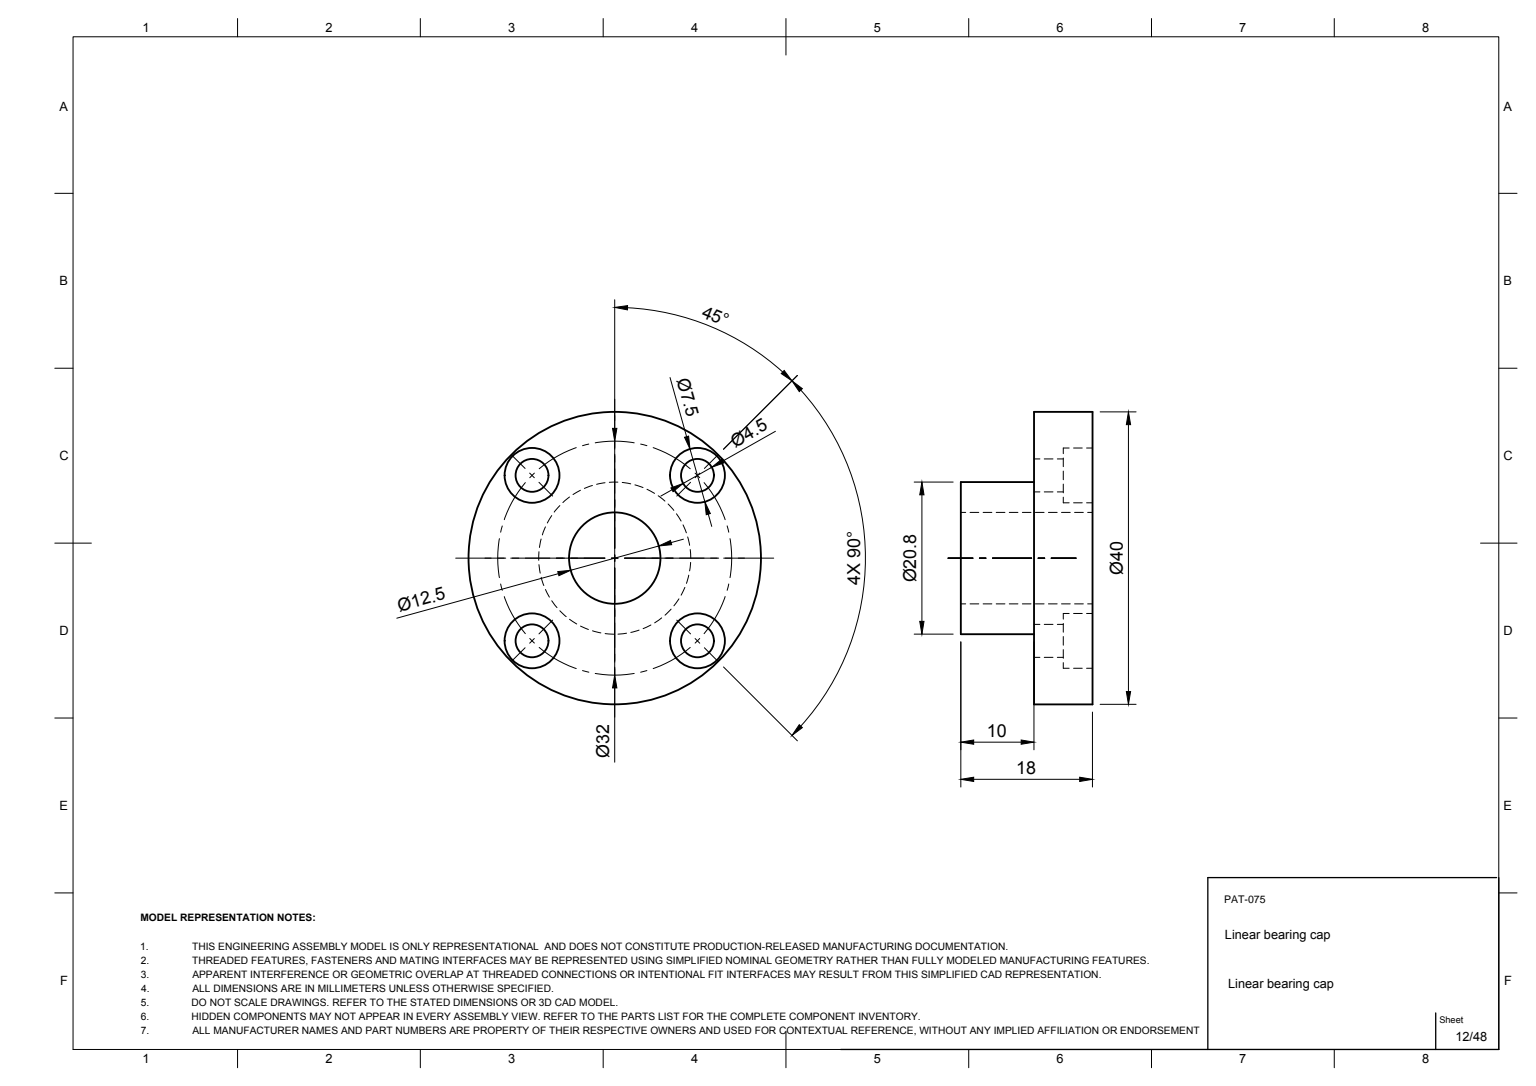
ISO-10303-21;
HEADER;
/* Generated by software containing ST-Developer
 * from STEP Tools, Inc. (www.steptools.com) 
 */

FILE_DESCRIPTION(
/* description */ ('Over-Centre Plunger Toggle Clamp on Slotted Fixture Frame'),
/* implementation_level */ '2;1');

FILE_NAME(
/* name */ 
'Linear bearing cap.step',
/* time_stamp */ '2026-10-28T03:23:24-07:00',
/* author */ (''),
/* organization */ (''),
/* preprocessor_version */ 'ST-DEVELOPER v20.2',
/* originating_system */ 'Autodesk Translation Framework v15.17.0.0',
/* authorisation */ '');

FILE_SCHEMA (('AUTOMOTIVE_DESIGN { 1 0 10303 214 3 1 1 }'));
ENDSEC;

DATA;
#10=MECHANICAL_DESIGN_GEOMETRIC_PRESENTATION_REPRESENTATION('',(#520),#15212);
#436=SHAPE_REPRESENTATION_RELATIONSHIP('SRR','None',#15410,#478);
#478=ADVANCED_BREP_SHAPE_REPRESENTATION('',(#571),#15172);
#520=STYLED_ITEM('',(#15719),#571);
#571=MANIFOLD_SOLID_BREP('Body1',#8252);
#693=FACE_BOUND('',#1755,.T.);
#694=FACE_BOUND('',#1758,.T.);
#695=FACE_BOUND('',#1761,.T.);
#696=FACE_BOUND('',#1764,.T.);
#697=FACE_BOUND('',#1771,.T.);
#698=FACE_BOUND('',#1775,.T.);
#699=FACE_BOUND('',#1776,.T.);
#700=FACE_BOUND('',#1777,.T.);
#701=FACE_BOUND('',#1778,.T.);
#702=FACE_BOUND('',#1779,.T.);
#703=FACE_BOUND('',#1781,.T.);
#704=FACE_BOUND('',#1782,.T.);
#705=FACE_BOUND('',#1783,.T.);
#706=FACE_BOUND('',#1784,.T.);
#707=FACE_BOUND('',#1785,.T.);
#833=PLANE('',#8970);
#834=PLANE('',#8975);
#835=PLANE('',#8980);
#836=PLANE('',#8985);
#837=PLANE('',#8998);
#838=PLANE('',#9005);
#839=PLANE('',#9006);
#1185=FACE_OUTER_BOUND('',#1753,.T.);
#1186=FACE_OUTER_BOUND('',#1754,.T.);
#1187=FACE_OUTER_BOUND('',#1756,.T.);
#1188=FACE_OUTER_BOUND('',#1757,.T.);
#1189=FACE_OUTER_BOUND('',#1759,.T.);
#1190=FACE_OUTER_BOUND('',#1760,.T.);
#1191=FACE_OUTER_BOUND('',#1762,.T.);
#1192=FACE_OUTER_BOUND('',#1763,.T.);
#1193=FACE_OUTER_BOUND('',#1765,.T.);
#1194=FACE_OUTER_BOUND('',#1766,.T.);
#1195=FACE_OUTER_BOUND('',#1767,.T.);
#1196=FACE_OUTER_BOUND('',#1768,.T.);
#1197=FACE_OUTER_BOUND('',#1769,.T.);
#1198=FACE_OUTER_BOUND('',#1770,.T.);
#1199=FACE_OUTER_BOUND('',#1772,.T.);
#1200=FACE_OUTER_BOUND('',#1773,.T.);
#1201=FACE_OUTER_BOUND('',#1774,.T.);
#1202=FACE_OUTER_BOUND('',#1780,.T.);
#1753=EDGE_LOOP('',(#6025,#6026,#6027,#6028));
#1754=EDGE_LOOP('',(#6029));
#1755=EDGE_LOOP('',(#6030));
#1756=EDGE_LOOP('',(#6031,#6032,#6033,#6034));
#1757=EDGE_LOOP('',(#6035));
#1758=EDGE_LOOP('',(#6036));
#1759=EDGE_LOOP('',(#6037,#6038,#6039,#6040));
#1760=EDGE_LOOP('',(#6041));
#1761=EDGE_LOOP('',(#6042));
#1762=EDGE_LOOP('',(#6043,#6044,#6045,#6046));
#1763=EDGE_LOOP('',(#6047));
#1764=EDGE_LOOP('',(#6048));
#1765=EDGE_LOOP('',(#6049,#6050,#6051,#6052));
#1766=EDGE_LOOP('',(#6053,#6054,#6055,#6056));
#1767=EDGE_LOOP('',(#6057,#6058,#6059,#6060));
#1768=EDGE_LOOP('',(#6061,#6062,#6063,#6064));
#1769=EDGE_LOOP('',(#6065,#6066,#6067,#6068));
#1770=EDGE_LOOP('',(#6069));
#1771=EDGE_LOOP('',(#6070));
#1772=EDGE_LOOP('',(#6071,#6072,#6073,#6074));
#1773=EDGE_LOOP('',(#6075,#6076,#6077,#6078));
#1774=EDGE_LOOP('',(#6079));
#1775=EDGE_LOOP('',(#6080));
#1776=EDGE_LOOP('',(#6081));
#1777=EDGE_LOOP('',(#6082));
#1778=EDGE_LOOP('',(#6083));
#1779=EDGE_LOOP('',(#6084));
#1780=EDGE_LOOP('',(#6085));
#1781=EDGE_LOOP('',(#6086));
#1782=EDGE_LOOP('',(#6087));
#1783=EDGE_LOOP('',(#6088));
#1784=EDGE_LOOP('',(#6089));
#1785=EDGE_LOOP('',(#6090));
#2363=LINE('',#12858,#2993);
#2364=LINE('',#12867,#2994);
#2365=LINE('',#12876,#2995);
#2366=LINE('',#12885,#2996);
#2367=LINE('',#12893,#2997);
#2368=LINE('',#12897,#2998);
#2369=LINE('',#12901,#2999);
#2370=LINE('',#12905,#3000);
#2371=LINE('',#12910,#3001);
#2372=LINE('',#12918,#3002);
#2373=LINE('',#12923,#3003);
#2993=VECTOR('',#10298,0.375);
#2994=VECTOR('',#10309,0.375);
#2995=VECTOR('',#10320,0.375);
#2996=VECTOR('',#10331,0.375);
#2997=VECTOR('',#10342,0.225);
#2998=VECTOR('',#10347,0.225);
#2999=VECTOR('',#10352,0.225);
#3000=VECTOR('',#10357,0.225);
#3001=VECTOR('',#10362,1.04);
#3002=VECTOR('',#10373,0.625);
#3003=VECTOR('',#10378,2.);
#3587=CIRCLE('',#8968,0.375);
#3588=CIRCLE('',#8969,0.375);
#3589=CIRCLE('',#8971,0.225);
#3590=CIRCLE('',#8973,0.375);
#3591=CIRCLE('',#8974,0.375);
#3592=CIRCLE('',#8976,0.225);
#3593=CIRCLE('',#8978,0.375);
#3594=CIRCLE('',#8979,0.375);
#3595=CIRCLE('',#8981,0.225);
#3596=CIRCLE('',#8983,0.375);
#3597=CIRCLE('',#8984,0.375);
#3598=CIRCLE('',#8986,0.225);
#3599=CIRCLE('',#8988,0.225);
#3600=CIRCLE('',#8990,0.225);
#3601=CIRCLE('',#8992,0.225);
#3602=CIRCLE('',#8994,0.225);
#3603=CIRCLE('',#8996,1.04);
#3604=CIRCLE('',#8997,1.04);
#3605=CIRCLE('',#8999,0.625);
#3606=CIRCLE('',#9001,0.625);
#3607=CIRCLE('',#9003,2.);
#3608=CIRCLE('',#9004,2.);
#4011=VERTEX_POINT('',#12855);
#4012=VERTEX_POINT('',#12857);
#4013=VERTEX_POINT('',#12861);
#4014=VERTEX_POINT('',#12864);
#4015=VERTEX_POINT('',#12866);
#4016=VERTEX_POINT('',#12870);
#4017=VERTEX_POINT('',#12873);
#4018=VERTEX_POINT('',#12875);
#4019=VERTEX_POINT('',#12879);
#4020=VERTEX_POINT('',#12882);
#4021=VERTEX_POINT('',#12884);
#4022=VERTEX_POINT('',#12888);
#4023=VERTEX_POINT('',#12891);
#4024=VERTEX_POINT('',#12895);
#4025=VERTEX_POINT('',#12899);
#4026=VERTEX_POINT('',#12903);
#4027=VERTEX_POINT('',#12907);
#4028=VERTEX_POINT('',#12909);
#4029=VERTEX_POINT('',#12913);
#4030=VERTEX_POINT('',#12916);
#4031=VERTEX_POINT('',#12920);
#4032=VERTEX_POINT('',#12922);
#4773=EDGE_CURVE('',#4011,#4011,#3587,.T.);
#4774=EDGE_CURVE('',#4011,#4012,#2363,.T.);
#4775=EDGE_CURVE('',#4012,#4012,#3588,.T.);
#4776=EDGE_CURVE('',#4013,#4013,#3589,.T.);
#4777=EDGE_CURVE('',#4014,#4014,#3590,.T.);
#4778=EDGE_CURVE('',#4014,#4015,#2364,.T.);
#4779=EDGE_CURVE('',#4015,#4015,#3591,.T.);
#4780=EDGE_CURVE('',#4016,#4016,#3592,.T.);
#4781=EDGE_CURVE('',#4017,#4017,#3593,.T.);
#4782=EDGE_CURVE('',#4017,#4018,#2365,.T.);
#4783=EDGE_CURVE('',#4018,#4018,#3594,.T.);
#4784=EDGE_CURVE('',#4019,#4019,#3595,.T.);
#4785=EDGE_CURVE('',#4020,#4020,#3596,.T.);
#4786=EDGE_CURVE('',#4020,#4021,#2366,.T.);
#4787=EDGE_CURVE('',#4021,#4021,#3597,.T.);
#4788=EDGE_CURVE('',#4022,#4022,#3598,.T.);
#4789=EDGE_CURVE('',#4023,#4023,#3599,.T.);
#4790=EDGE_CURVE('',#4023,#4013,#2367,.T.);
#4791=EDGE_CURVE('',#4024,#4024,#3600,.T.);
#4792=EDGE_CURVE('',#4024,#4016,#2368,.T.);
#4793=EDGE_CURVE('',#4025,#4025,#3601,.T.);
#4794=EDGE_CURVE('',#4025,#4019,#2369,.T.);
#4795=EDGE_CURVE('',#4026,#4026,#3602,.T.);
#4796=EDGE_CURVE('',#4026,#4022,#2370,.T.);
#4797=EDGE_CURVE('',#4027,#4027,#3603,.T.);
#4798=EDGE_CURVE('',#4027,#4028,#2371,.T.);
#4799=EDGE_CURVE('',#4028,#4028,#3604,.T.);
#4800=EDGE_CURVE('',#4029,#4029,#3605,.T.);
#4801=EDGE_CURVE('',#4030,#4030,#3606,.T.);
#4802=EDGE_CURVE('',#4030,#4029,#2372,.T.);
#4803=EDGE_CURVE('',#4031,#4031,#3607,.T.);
#4804=EDGE_CURVE('',#4031,#4032,#2373,.T.);
#4805=EDGE_CURVE('',#4032,#4032,#3608,.T.);
#6025=ORIENTED_EDGE('',*,*,#4773,.F.);
#6026=ORIENTED_EDGE('',*,*,#4774,.T.);
#6027=ORIENTED_EDGE('',*,*,#4775,.F.);
#6028=ORIENTED_EDGE('',*,*,#4774,.F.);
#6029=ORIENTED_EDGE('',*,*,#4773,.T.);
#6030=ORIENTED_EDGE('',*,*,#4776,.F.);
#6031=ORIENTED_EDGE('',*,*,#4777,.F.);
#6032=ORIENTED_EDGE('',*,*,#4778,.T.);
#6033=ORIENTED_EDGE('',*,*,#4779,.F.);
#6034=ORIENTED_EDGE('',*,*,#4778,.F.);
#6035=ORIENTED_EDGE('',*,*,#4777,.T.);
#6036=ORIENTED_EDGE('',*,*,#4780,.F.);
#6037=ORIENTED_EDGE('',*,*,#4781,.F.);
#6038=ORIENTED_EDGE('',*,*,#4782,.T.);
#6039=ORIENTED_EDGE('',*,*,#4783,.F.);
#6040=ORIENTED_EDGE('',*,*,#4782,.F.);
#6041=ORIENTED_EDGE('',*,*,#4781,.T.);
#6042=ORIENTED_EDGE('',*,*,#4784,.F.);
#6043=ORIENTED_EDGE('',*,*,#4785,.F.);
#6044=ORIENTED_EDGE('',*,*,#4786,.T.);
#6045=ORIENTED_EDGE('',*,*,#4787,.F.);
#6046=ORIENTED_EDGE('',*,*,#4786,.F.);
#6047=ORIENTED_EDGE('',*,*,#4785,.T.);
#6048=ORIENTED_EDGE('',*,*,#4788,.F.);
#6049=ORIENTED_EDGE('',*,*,#4789,.F.);
#6050=ORIENTED_EDGE('',*,*,#4790,.T.);
#6051=ORIENTED_EDGE('',*,*,#4776,.T.);
#6052=ORIENTED_EDGE('',*,*,#4790,.F.);
#6053=ORIENTED_EDGE('',*,*,#4791,.F.);
#6054=ORIENTED_EDGE('',*,*,#4792,.T.);
#6055=ORIENTED_EDGE('',*,*,#4780,.T.);
#6056=ORIENTED_EDGE('',*,*,#4792,.F.);
#6057=ORIENTED_EDGE('',*,*,#4793,.F.);
#6058=ORIENTED_EDGE('',*,*,#4794,.T.);
#6059=ORIENTED_EDGE('',*,*,#4784,.T.);
#6060=ORIENTED_EDGE('',*,*,#4794,.F.);
#6061=ORIENTED_EDGE('',*,*,#4795,.F.);
#6062=ORIENTED_EDGE('',*,*,#4796,.T.);
#6063=ORIENTED_EDGE('',*,*,#4788,.T.);
#6064=ORIENTED_EDGE('',*,*,#4796,.F.);
#6065=ORIENTED_EDGE('',*,*,#4797,.F.);
#6066=ORIENTED_EDGE('',*,*,#4798,.T.);
#6067=ORIENTED_EDGE('',*,*,#4799,.T.);
#6068=ORIENTED_EDGE('',*,*,#4798,.F.);
#6069=ORIENTED_EDGE('',*,*,#4799,.F.);
#6070=ORIENTED_EDGE('',*,*,#4800,.F.);
#6071=ORIENTED_EDGE('',*,*,#4801,.F.);
#6072=ORIENTED_EDGE('',*,*,#4802,.T.);
#6073=ORIENTED_EDGE('',*,*,#4800,.T.);
#6074=ORIENTED_EDGE('',*,*,#4802,.F.);
#6075=ORIENTED_EDGE('',*,*,#4803,.F.);
#6076=ORIENTED_EDGE('',*,*,#4804,.T.);
#6077=ORIENTED_EDGE('',*,*,#4805,.T.);
#6078=ORIENTED_EDGE('',*,*,#4804,.F.);
#6079=ORIENTED_EDGE('',*,*,#4803,.T.);
#6080=ORIENTED_EDGE('',*,*,#4801,.T.);
#6081=ORIENTED_EDGE('',*,*,#4787,.T.);
#6082=ORIENTED_EDGE('',*,*,#4783,.T.);
#6083=ORIENTED_EDGE('',*,*,#4779,.T.);
#6084=ORIENTED_EDGE('',*,*,#4775,.T.);
#6085=ORIENTED_EDGE('',*,*,#4805,.F.);
#6086=ORIENTED_EDGE('',*,*,#4797,.T.);
#6087=ORIENTED_EDGE('',*,*,#4795,.T.);
#6088=ORIENTED_EDGE('',*,*,#4793,.T.);
#6089=ORIENTED_EDGE('',*,*,#4791,.T.);
#6090=ORIENTED_EDGE('',*,*,#4789,.T.);
#7665=CYLINDRICAL_SURFACE('',#8967,0.375);
#7666=CYLINDRICAL_SURFACE('',#8972,0.375);
#7667=CYLINDRICAL_SURFACE('',#8977,0.375);
#7668=CYLINDRICAL_SURFACE('',#8982,0.375);
#7669=CYLINDRICAL_SURFACE('',#8987,0.225);
#7670=CYLINDRICAL_SURFACE('',#8989,0.225);
#7671=CYLINDRICAL_SURFACE('',#8991,0.225);
#7672=CYLINDRICAL_SURFACE('',#8993,0.225);
#7673=CYLINDRICAL_SURFACE('',#8995,1.04);
#7674=CYLINDRICAL_SURFACE('',#9000,0.625);
#7675=CYLINDRICAL_SURFACE('',#9002,2.);
#7857=ADVANCED_FACE('',(#1185),#7665,.F.);
#7858=ADVANCED_FACE('',(#1186,#693),#833,.T.);
#7859=ADVANCED_FACE('',(#1187),#7666,.F.);
#7860=ADVANCED_FACE('',(#1188,#694),#834,.T.);
#7861=ADVANCED_FACE('',(#1189),#7667,.F.);
#7862=ADVANCED_FACE('',(#1190,#695),#835,.T.);
#7863=ADVANCED_FACE('',(#1191),#7668,.F.);
#7864=ADVANCED_FACE('',(#1192,#696),#836,.T.);
#7865=ADVANCED_FACE('',(#1193),#7669,.F.);
#7866=ADVANCED_FACE('',(#1194),#7670,.F.);
#7867=ADVANCED_FACE('',(#1195),#7671,.F.);
#7868=ADVANCED_FACE('',(#1196),#7672,.F.);
#7869=ADVANCED_FACE('',(#1197),#7673,.T.);
#7870=ADVANCED_FACE('',(#1198,#697),#837,.F.);
#7871=ADVANCED_FACE('',(#1199),#7674,.F.);
#7872=ADVANCED_FACE('',(#1200),#7675,.T.);
#7873=ADVANCED_FACE('',(#1201,#698,#699,#700,#701,#702),#838,.T.);
#7874=ADVANCED_FACE('',(#1202,#703,#704,#705,#706,#707),#839,.F.);
#8252=CLOSED_SHELL('',(#7857,#7858,#7859,#7860,#7861,#7862,#7863,#7864,
#7865,#7866,#7867,#7868,#7869,#7870,#7871,#7872,#7873,#7874));
#8966=AXIS2_PLACEMENT_3D('',#12853,#10292,#10293);
#8967=AXIS2_PLACEMENT_3D('',#12854,#10294,#10295);
#8968=AXIS2_PLACEMENT_3D('',#12856,#10296,#10297);
#8969=AXIS2_PLACEMENT_3D('',#12859,#10299,#10300);
#8970=AXIS2_PLACEMENT_3D('',#12860,#10301,#10302);
#8971=AXIS2_PLACEMENT_3D('',#12862,#10303,#10304);
#8972=AXIS2_PLACEMENT_3D('',#12863,#10305,#10306);
#8973=AXIS2_PLACEMENT_3D('',#12865,#10307,#10308);
#8974=AXIS2_PLACEMENT_3D('',#12868,#10310,#10311);
#8975=AXIS2_PLACEMENT_3D('',#12869,#10312,#10313);
#8976=AXIS2_PLACEMENT_3D('',#12871,#10314,#10315);
#8977=AXIS2_PLACEMENT_3D('',#12872,#10316,#10317);
#8978=AXIS2_PLACEMENT_3D('',#12874,#10318,#10319);
#8979=AXIS2_PLACEMENT_3D('',#12877,#10321,#10322);
#8980=AXIS2_PLACEMENT_3D('',#12878,#10323,#10324);
#8981=AXIS2_PLACEMENT_3D('',#12880,#10325,#10326);
#8982=AXIS2_PLACEMENT_3D('',#12881,#10327,#10328);
#8983=AXIS2_PLACEMENT_3D('',#12883,#10329,#10330);
#8984=AXIS2_PLACEMENT_3D('',#12886,#10332,#10333);
#8985=AXIS2_PLACEMENT_3D('',#12887,#10334,#10335);
#8986=AXIS2_PLACEMENT_3D('',#12889,#10336,#10337);
#8987=AXIS2_PLACEMENT_3D('',#12890,#10338,#10339);
#8988=AXIS2_PLACEMENT_3D('',#12892,#10340,#10341);
#8989=AXIS2_PLACEMENT_3D('',#12894,#10343,#10344);
#8990=AXIS2_PLACEMENT_3D('',#12896,#10345,#10346);
#8991=AXIS2_PLACEMENT_3D('',#12898,#10348,#10349);
#8992=AXIS2_PLACEMENT_3D('',#12900,#10350,#10351);
#8993=AXIS2_PLACEMENT_3D('',#12902,#10353,#10354);
#8994=AXIS2_PLACEMENT_3D('',#12904,#10355,#10356);
#8995=AXIS2_PLACEMENT_3D('',#12906,#10358,#10359);
#8996=AXIS2_PLACEMENT_3D('',#12908,#10360,#10361);
#8997=AXIS2_PLACEMENT_3D('',#12911,#10363,#10364);
#8998=AXIS2_PLACEMENT_3D('',#12912,#10365,#10366);
#8999=AXIS2_PLACEMENT_3D('',#12914,#10367,#10368);
#9000=AXIS2_PLACEMENT_3D('',#12915,#10369,#10370);
#9001=AXIS2_PLACEMENT_3D('',#12917,#10371,#10372);
#9002=AXIS2_PLACEMENT_3D('',#12919,#10374,#10375);
#9003=AXIS2_PLACEMENT_3D('',#12921,#10376,#10377);
#9004=AXIS2_PLACEMENT_3D('',#12924,#10379,#10380);
#9005=AXIS2_PLACEMENT_3D('',#12925,#10381,#10382);
#9006=AXIS2_PLACEMENT_3D('',#12926,#10383,#10384);
#10292=DIRECTION('axis',(0.,0.,1.));
#10293=DIRECTION('refdir',(1.,0.,0.));
#10294=DIRECTION('center_axis',(0.,0.,1.));
#10295=DIRECTION('ref_axis',(1.,0.,0.));
#10296=DIRECTION('center_axis',(0.,0.,1.));
#10297=DIRECTION('ref_axis',(1.,0.,0.));
#10298=DIRECTION('',(0.,0.,1.));
#10299=DIRECTION('center_axis',(0.,0.,-1.));
#10300=DIRECTION('ref_axis',(1.,0.,0.));
#10301=DIRECTION('center_axis',(0.,0.,1.));
#10302=DIRECTION('ref_axis',(1.,0.,0.));
#10303=DIRECTION('center_axis',(0.,0.,1.));
#10304=DIRECTION('ref_axis',(1.,0.,0.));
#10305=DIRECTION('center_axis',(0.,0.,1.));
#10306=DIRECTION('ref_axis',(1.,0.,0.));
#10307=DIRECTION('center_axis',(0.,0.,1.));
#10308=DIRECTION('ref_axis',(1.,0.,0.));
#10309=DIRECTION('',(0.,0.,1.));
#10310=DIRECTION('center_axis',(0.,0.,-1.));
#10311=DIRECTION('ref_axis',(1.,0.,0.));
#10312=DIRECTION('center_axis',(0.,0.,1.));
#10313=DIRECTION('ref_axis',(1.,0.,0.));
#10314=DIRECTION('center_axis',(0.,0.,1.));
#10315=DIRECTION('ref_axis',(1.,0.,0.));
#10316=DIRECTION('center_axis',(0.,0.,1.));
#10317=DIRECTION('ref_axis',(1.,0.,0.));
#10318=DIRECTION('center_axis',(0.,0.,1.));
#10319=DIRECTION('ref_axis',(1.,0.,0.));
#10320=DIRECTION('',(0.,0.,1.));
#10321=DIRECTION('center_axis',(0.,0.,-1.));
#10322=DIRECTION('ref_axis',(1.,0.,0.));
#10323=DIRECTION('center_axis',(0.,0.,1.));
#10324=DIRECTION('ref_axis',(1.,0.,0.));
#10325=DIRECTION('center_axis',(0.,0.,1.));
#10326=DIRECTION('ref_axis',(1.,0.,0.));
#10327=DIRECTION('center_axis',(0.,0.,1.));
#10328=DIRECTION('ref_axis',(1.,0.,0.));
#10329=DIRECTION('center_axis',(0.,0.,1.));
#10330=DIRECTION('ref_axis',(1.,0.,0.));
#10331=DIRECTION('',(0.,0.,1.));
#10332=DIRECTION('center_axis',(0.,0.,-1.));
#10333=DIRECTION('ref_axis',(1.,0.,0.));
#10334=DIRECTION('center_axis',(0.,0.,1.));
#10335=DIRECTION('ref_axis',(1.,0.,0.));
#10336=DIRECTION('center_axis',(0.,0.,1.));
#10337=DIRECTION('ref_axis',(1.,0.,0.));
#10338=DIRECTION('center_axis',(0.,0.,1.));
#10339=DIRECTION('ref_axis',(1.,0.,0.));
#10340=DIRECTION('center_axis',(0.,0.,1.));
#10341=DIRECTION('ref_axis',(1.,0.,0.));
#10342=DIRECTION('',(0.,0.,1.));
#10343=DIRECTION('center_axis',(0.,0.,1.));
#10344=DIRECTION('ref_axis',(1.,0.,0.));
#10345=DIRECTION('center_axis',(0.,0.,1.));
#10346=DIRECTION('ref_axis',(1.,0.,0.));
#10347=DIRECTION('',(0.,0.,1.));
#10348=DIRECTION('center_axis',(0.,0.,1.));
#10349=DIRECTION('ref_axis',(1.,0.,0.));
#10350=DIRECTION('center_axis',(0.,0.,1.));
#10351=DIRECTION('ref_axis',(1.,0.,0.));
#10352=DIRECTION('',(0.,0.,1.));
#10353=DIRECTION('center_axis',(0.,0.,1.));
#10354=DIRECTION('ref_axis',(1.,0.,0.));
#10355=DIRECTION('center_axis',(0.,0.,1.));
#10356=DIRECTION('ref_axis',(1.,0.,0.));
#10357=DIRECTION('',(0.,0.,1.));
#10358=DIRECTION('center_axis',(0.,0.,1.));
#10359=DIRECTION('ref_axis',(1.,0.,0.));
#10360=DIRECTION('center_axis',(0.,0.,1.));
#10361=DIRECTION('ref_axis',(1.,0.,0.));
#10362=DIRECTION('',(0.,0.,-1.));
#10363=DIRECTION('center_axis',(0.,0.,1.));
#10364=DIRECTION('ref_axis',(1.,0.,0.));
#10365=DIRECTION('center_axis',(0.,0.,1.));
#10366=DIRECTION('ref_axis',(1.,0.,0.));
#10367=DIRECTION('center_axis',(0.,0.,-1.));
#10368=DIRECTION('ref_axis',(1.,0.,0.));
#10369=DIRECTION('center_axis',(0.,0.,1.));
#10370=DIRECTION('ref_axis',(1.,0.,0.));
#10371=DIRECTION('center_axis',(0.,0.,-1.));
#10372=DIRECTION('ref_axis',(1.,0.,0.));
#10373=DIRECTION('',(0.,0.,-1.));
#10374=DIRECTION('center_axis',(0.,0.,1.));
#10375=DIRECTION('ref_axis',(1.,0.,0.));
#10376=DIRECTION('center_axis',(0.,0.,1.));
#10377=DIRECTION('ref_axis',(1.,0.,0.));
#10378=DIRECTION('',(0.,0.,-1.));
#10379=DIRECTION('center_axis',(0.,0.,1.));
#10380=DIRECTION('ref_axis',(1.,0.,0.));
#10381=DIRECTION('center_axis',(0.,0.,1.));
#10382=DIRECTION('ref_axis',(1.,0.,0.));
#10383=DIRECTION('center_axis',(0.,0.,1.));
#10384=DIRECTION('ref_axis',(1.,0.,0.));
#12853=CARTESIAN_POINT('',(0.,0.,0.));
#12854=CARTESIAN_POINT('Origin',(-1.13137084989848,-1.13137084989848,16.9));
#12855=CARTESIAN_POINT('',(-1.50637084989848,-1.13137084989848,16.9));
#12856=CARTESIAN_POINT('Origin',(-1.13137084989848,-1.13137084989848,16.9));
#12857=CARTESIAN_POINT('',(-1.50637084989848,-1.13137084989848,17.3));
#12858=CARTESIAN_POINT('',(-1.50637084989848,-1.13137084989848,16.9));
#12859=CARTESIAN_POINT('Origin',(-1.13137084989848,-1.13137084989848,17.3));
#12860=CARTESIAN_POINT('Origin',(-1.13137084989848,-1.13137084989848,16.9));
#12861=CARTESIAN_POINT('',(-1.35637084989848,-1.13137084989848,16.9));
#12862=CARTESIAN_POINT('Origin',(-1.13137084989848,-1.13137084989848,16.9));
#12863=CARTESIAN_POINT('Origin',(-1.13137084989848,1.13137084989848,16.9));
#12864=CARTESIAN_POINT('',(-1.50637084989848,1.13137084989848,16.9));
#12865=CARTESIAN_POINT('Origin',(-1.13137084989848,1.13137084989848,16.9));
#12866=CARTESIAN_POINT('',(-1.50637084989848,1.13137084989848,17.3));
#12867=CARTESIAN_POINT('',(-1.50637084989848,1.13137084989848,16.9));
#12868=CARTESIAN_POINT('Origin',(-1.13137084989848,1.13137084989848,17.3));
#12869=CARTESIAN_POINT('Origin',(-1.13137084989848,1.13137084989848,16.9));
#12870=CARTESIAN_POINT('',(-1.35637084989848,1.13137084989848,16.9));
#12871=CARTESIAN_POINT('Origin',(-1.13137084989848,1.13137084989848,16.9));
#12872=CARTESIAN_POINT('Origin',(1.13137084989848,1.13137084989848,16.9));
#12873=CARTESIAN_POINT('',(0.756370849898476,1.13137084989848,16.9));
#12874=CARTESIAN_POINT('Origin',(1.13137084989848,1.13137084989848,16.9));
#12875=CARTESIAN_POINT('',(0.756370849898476,1.13137084989848,17.3));
#12876=CARTESIAN_POINT('',(0.756370849898476,1.13137084989848,16.9));
#12877=CARTESIAN_POINT('Origin',(1.13137084989848,1.13137084989848,17.3));
#12878=CARTESIAN_POINT('Origin',(1.13137084989848,1.13137084989848,16.9));
#12879=CARTESIAN_POINT('',(0.906370849898476,1.13137084989848,16.9));
#12880=CARTESIAN_POINT('Origin',(1.13137084989848,1.13137084989848,16.9));
#12881=CARTESIAN_POINT('Origin',(1.13137084989848,-1.13137084989848,16.9));
#12882=CARTESIAN_POINT('',(0.756370849898476,-1.13137084989848,16.9));
#12883=CARTESIAN_POINT('Origin',(1.13137084989848,-1.13137084989848,16.9));
#12884=CARTESIAN_POINT('',(0.756370849898476,-1.13137084989848,17.3));
#12885=CARTESIAN_POINT('',(0.756370849898476,-1.13137084989848,16.9));
#12886=CARTESIAN_POINT('Origin',(1.13137084989848,-1.13137084989848,17.3));
#12887=CARTESIAN_POINT('Origin',(1.13137084989848,-1.13137084989848,16.9));
#12888=CARTESIAN_POINT('',(0.906370849898476,-1.13137084989848,16.9));
#12889=CARTESIAN_POINT('Origin',(1.13137084989848,-1.13137084989848,16.9));
#12890=CARTESIAN_POINT('Origin',(-1.13137084989848,-1.13137084989848,16.4));
#12891=CARTESIAN_POINT('',(-1.35637084989848,-1.13137084989848,16.5));
#12892=CARTESIAN_POINT('Origin',(-1.13137084989848,-1.13137084989848,16.5));
#12893=CARTESIAN_POINT('',(-1.35637084989848,-1.13137084989848,16.4));
#12894=CARTESIAN_POINT('Origin',(-1.13137084989848,1.13137084989848,16.4));
#12895=CARTESIAN_POINT('',(-1.35637084989848,1.13137084989848,16.5));
#12896=CARTESIAN_POINT('Origin',(-1.13137084989848,1.13137084989848,16.5));
#12897=CARTESIAN_POINT('',(-1.35637084989848,1.13137084989848,16.4));
#12898=CARTESIAN_POINT('Origin',(1.13137084989848,1.13137084989848,16.4));
#12899=CARTESIAN_POINT('',(0.906370849898476,1.13137084989848,16.5));
#12900=CARTESIAN_POINT('Origin',(1.13137084989848,1.13137084989848,16.5));
#12901=CARTESIAN_POINT('',(0.906370849898476,1.13137084989848,16.4));
#12902=CARTESIAN_POINT('Origin',(1.13137084989848,-1.13137084989848,16.4));
#12903=CARTESIAN_POINT('',(0.906370849898476,-1.13137084989848,16.5));
#12904=CARTESIAN_POINT('Origin',(1.13137084989848,-1.13137084989848,16.5));
#12905=CARTESIAN_POINT('',(0.906370849898476,-1.13137084989848,16.4));
#12906=CARTESIAN_POINT('Origin',(0.,0.,15.5));
#12907=CARTESIAN_POINT('',(-1.04,-1.27363267111325E-16,16.5));
#12908=CARTESIAN_POINT('Origin',(0.,0.,16.5));
#12909=CARTESIAN_POINT('',(-1.04,-1.27363267111325E-16,15.5));
#12910=CARTESIAN_POINT('',(-1.04,-1.27363267111325E-16,15.5));
#12911=CARTESIAN_POINT('Origin',(0.,0.,15.5));
#12912=CARTESIAN_POINT('Origin',(0.,0.,15.5));
#12913=CARTESIAN_POINT('',(-0.625,-7.65404249467096E-17,15.5));
#12914=CARTESIAN_POINT('Origin',(0.,0.,15.5));
#12915=CARTESIAN_POINT('Origin',(0.,0.,16.5));
#12916=CARTESIAN_POINT('',(-0.625,-7.65404249467096E-17,17.3));
#12917=CARTESIAN_POINT('Origin',(0.,0.,17.3));
#12918=CARTESIAN_POINT('',(-0.625,-7.65404249467096E-17,16.5));
#12919=CARTESIAN_POINT('Origin',(0.,0.,16.5));
#12920=CARTESIAN_POINT('',(-2.,-2.44929359829471E-16,17.3));
#12921=CARTESIAN_POINT('Origin',(0.,0.,17.3));
#12922=CARTESIAN_POINT('',(-2.,-2.44929359829471E-16,16.5));
#12923=CARTESIAN_POINT('',(-2.,-2.44929359829471E-16,16.5));
#12924=CARTESIAN_POINT('Origin',(0.,0.,16.5));
#12925=CARTESIAN_POINT('Origin',(0.,0.,17.3));
#12926=CARTESIAN_POINT('Origin',(0.,0.,16.5));
#15122=UNCERTAINTY_MEASURE_WITH_UNIT(LENGTH_MEASURE(0.001),#15213,
'DISTANCE_ACCURACY_VALUE',
'Maximum model space distance between geometric entities at asserted c
onnectivities');
#15162=UNCERTAINTY_MEASURE_WITH_UNIT(LENGTH_MEASURE(0.001),#15213,
'DISTANCE_ACCURACY_VALUE',
'Maximum model space distance between geometric entities at asserted c
onnectivities');
#15172=(
GEOMETRIC_REPRESENTATION_CONTEXT(3)
GLOBAL_UNCERTAINTY_ASSIGNED_CONTEXT((#15122))
GLOBAL_UNIT_ASSIGNED_CONTEXT((#15213,#15215,#15216))
REPRESENTATION_CONTEXT('','3D')
);
#15212=(
GEOMETRIC_REPRESENTATION_CONTEXT(3)
GLOBAL_UNCERTAINTY_ASSIGNED_CONTEXT((#15162))
GLOBAL_UNIT_ASSIGNED_CONTEXT((#15213,#15215,#15216))
REPRESENTATION_CONTEXT('','3D')
);
#15213=(
LENGTH_UNIT()
NAMED_UNIT(*)
SI_UNIT(.CENTI.,.METRE.)
);
#15215=(
NAMED_UNIT(*)
PLANE_ANGLE_UNIT()
SI_UNIT($,.RADIAN.)
);
#15216=(
NAMED_UNIT(*)
SI_UNIT($,.STERADIAN.)
SOLID_ANGLE_UNIT()
);
#15226=SHAPE_DEFINITION_REPRESENTATION(#15275,#15410);
#15275=PRODUCT_DEFINITION_SHAPE('',$,#15460);
#15410=SHAPE_REPRESENTATION('',(#8966),#15172);
#15450=PRODUCT_DEFINITION_CONTEXT('part definition',#15599,'design');
#15460=PRODUCT_DEFINITION('Linear bearing cap','Linear bearing cap',#15509,
#15450);
#15509=PRODUCT_DEFINITION_FORMATION('',$,#15610);
#15599=APPLICATION_CONTEXT(
'Core Data for Automotive Mechanical Design Process');
#15600=PRODUCT_CONTEXT('part definition',#15599,'mechanical');
#15610=PRODUCT('Linear bearing cap','Linear bearing cap',
'Linear bearing cap',(#15600));
#15713=COLOUR_RGB('Grey',0.48,0.52,0.57);
#15714=FILL_AREA_STYLE_COLOUR('',#15713);
#15715=FILL_AREA_STYLE('',(#15714));
#15716=SURFACE_STYLE_FILL_AREA(#15715);
#15717=SURFACE_SIDE_STYLE('',(#15716));
#15718=SURFACE_STYLE_USAGE(.BOTH.,#15717);
#15719=PRESENTATION_STYLE_ASSIGNMENT((#15718));
ENDSEC;
END-ISO-10303-21;
